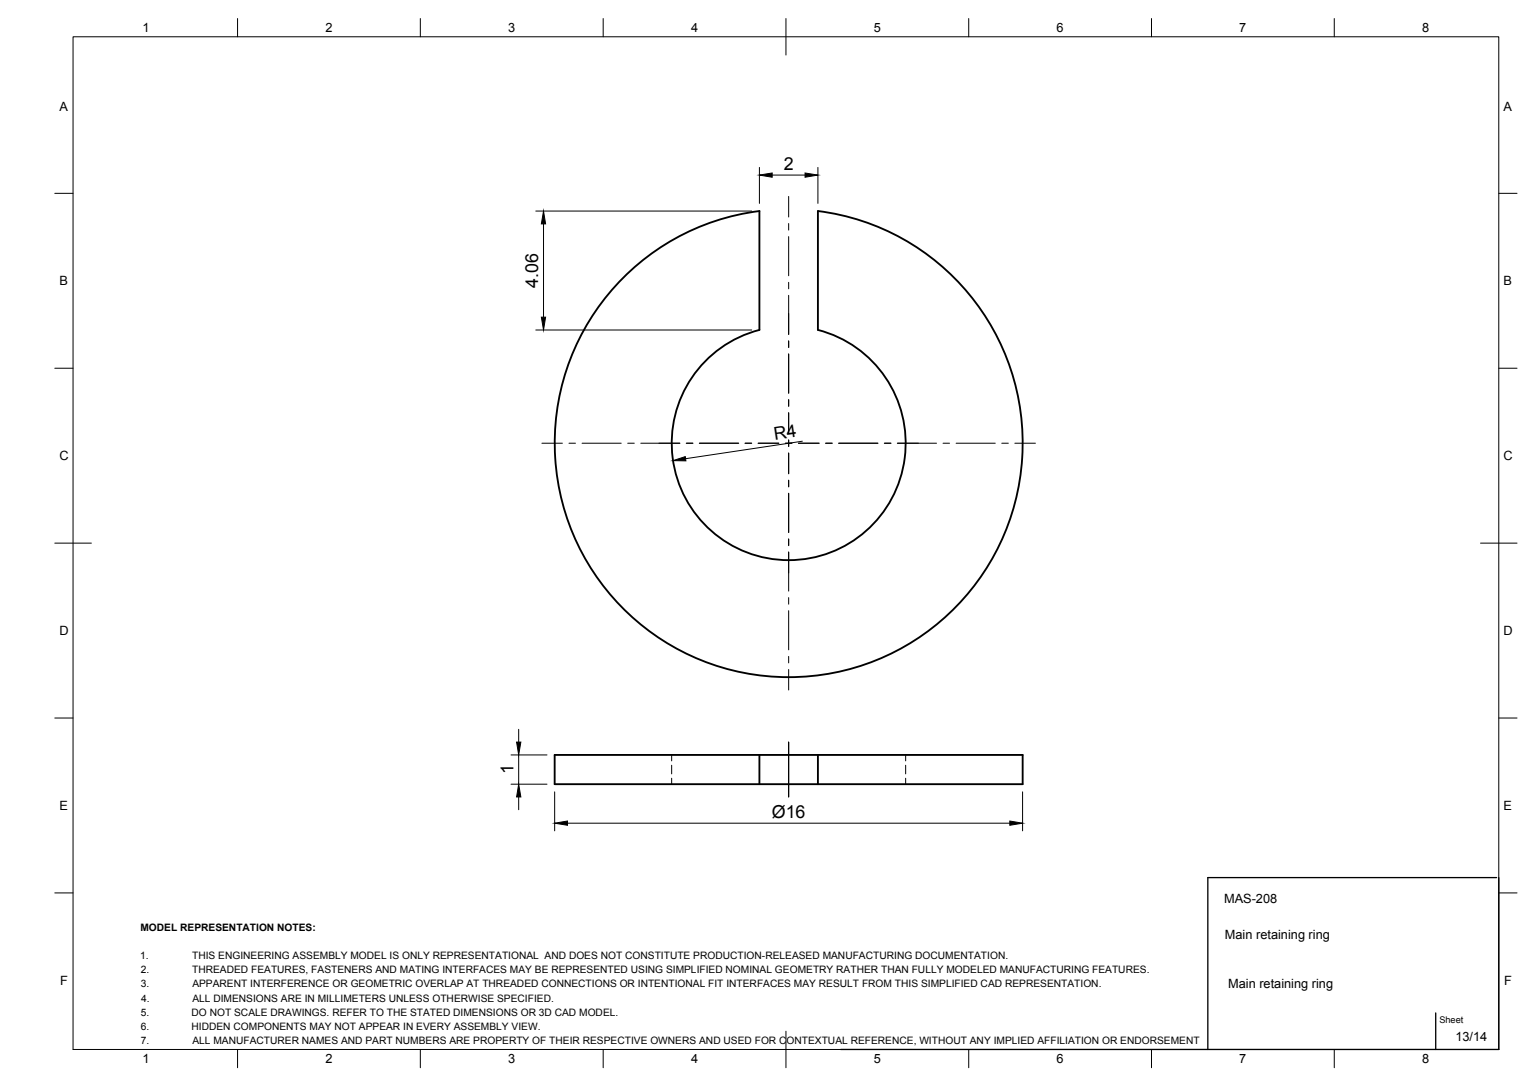
ISO-10303-21;
HEADER;
/* Generated by software containing ST-Developer
 * from STEP Tools, Inc. (www.steptools.com) 
 */

FILE_DESCRIPTION(
/* description */ ('Independent vertical20-tooth ratchet advance with repeated integral-c
ounterweight gravity pawls, swinging drive lever, bronze sleeves and f
ully retained axle stacks.18degpertooth. Native revolutes; geometric c
ycle checking rather than automatic contact/rolling dynamics. Gravity 
closing checked from actual pawl center of mass. Backplate/foot suppor
ts unit. Fits, torque, holding force, wear and life unassigned.'),
/* implementation_level */ '2;1');

FILE_NAME(
/* name */ 'Main retaining ring.step',
/* time_stamp */ '2026-11-09T06:25:53-08:00',
/* author */ (''),
/* organization */ (''),
/* preprocessor_version */ 'ST-DEVELOPER v20.2',
/* originating_system */ 'Autodesk Translation Framework v15.17.0.0',
/* authorisation */ '');

FILE_SCHEMA (('AUTOMOTIVE_DESIGN { 1 0 10303 214 3 1 1 }'));
ENDSEC;

DATA;
#10=MECHANICAL_DESIGN_GEOMETRIC_PRESENTATION_REPRESENTATION('',(#129),#4643);
#101=SHAPE_REPRESENTATION_RELATIONSHIP('SRR','None',#4706,#115);
#115=ADVANCED_BREP_SHAPE_REPRESENTATION('',(#143),#4635);
#129=STYLED_ITEM('',(#4783),#143);
#143=MANIFOLD_SOLID_BREP('Body1',#2665);
#269=PLANE('',#2979);
#270=PLANE('',#2980);
#271=PLANE('',#2981);
#272=PLANE('',#2988);
#403=FACE_OUTER_BOUND('',#581,.T.);
#404=FACE_OUTER_BOUND('',#582,.T.);
#405=FACE_OUTER_BOUND('',#583,.T.);
#406=FACE_OUTER_BOUND('',#584,.T.);
#407=FACE_OUTER_BOUND('',#585,.T.);
#408=FACE_OUTER_BOUND('',#586,.T.);
#581=EDGE_LOOP('',(#2269,#2270,#2271,#2272));
#582=EDGE_LOOP('',(#2273,#2274,#2275,#2276));
#583=EDGE_LOOP('',(#2277,#2278,#2279,#2280));
#584=EDGE_LOOP('',(#2281,#2282,#2283,#2284));
#585=EDGE_LOOP('',(#2285,#2286,#2287,#2288));
#586=EDGE_LOOP('',(#2289,#2290,#2291,#2292));
#833=LINE('',#4367,#1095);
#834=LINE('',#4369,#1096);
#835=LINE('',#4371,#1097);
#836=LINE('',#4372,#1098);
#837=LINE('',#4376,#1099);
#838=LINE('',#4378,#1100);
#839=LINE('',#4380,#1101);
#840=LINE('',#4381,#1102);
#1095=VECTOR('',#3581,10.);
#1096=VECTOR('',#3582,10.);
#1097=VECTOR('',#3583,10.);
#1098=VECTOR('',#3584,10.);
#1099=VECTOR('',#3587,10.);
#1100=VECTOR('',#3588,10.);
#1101=VECTOR('',#3589,10.);
#1102=VECTOR('',#3590,10.);
#1211=CIRCLE('',#2982,8.);
#1212=CIRCLE('',#2983,4.);
#1213=CIRCLE('',#2985,4.);
#1214=CIRCLE('',#2987,8.);
#1397=VERTEX_POINT('',#4365);
#1398=VERTEX_POINT('',#4366);
#1399=VERTEX_POINT('',#4368);
#1400=VERTEX_POINT('',#4370);
#1401=VERTEX_POINT('',#4374);
#1402=VERTEX_POINT('',#4375);
#1403=VERTEX_POINT('',#4377);
#1404=VERTEX_POINT('',#4379);
#1699=EDGE_CURVE('',#1397,#1398,#833,.T.);
#1700=EDGE_CURVE('',#1399,#1397,#834,.T.);
#1701=EDGE_CURVE('',#1400,#1399,#835,.T.);
#1702=EDGE_CURVE('',#1398,#1400,#836,.T.);
#1703=EDGE_CURVE('',#1401,#1402,#837,.T.);
#1704=EDGE_CURVE('',#1403,#1401,#838,.T.);
#1705=EDGE_CURVE('',#1404,#1403,#839,.T.);
#1706=EDGE_CURVE('',#1402,#1404,#840,.T.);
#1707=EDGE_CURVE('',#1399,#1404,#1211,.T.);
#1708=EDGE_CURVE('',#1402,#1397,#1212,.T.);
#1709=EDGE_CURVE('',#1401,#1398,#1213,.T.);
#1710=EDGE_CURVE('',#1400,#1403,#1214,.T.);
#2269=ORIENTED_EDGE('',*,*,#1699,.F.);
#2270=ORIENTED_EDGE('',*,*,#1700,.F.);
#2271=ORIENTED_EDGE('',*,*,#1701,.F.);
#2272=ORIENTED_EDGE('',*,*,#1702,.F.);
#2273=ORIENTED_EDGE('',*,*,#1703,.F.);
#2274=ORIENTED_EDGE('',*,*,#1704,.F.);
#2275=ORIENTED_EDGE('',*,*,#1705,.F.);
#2276=ORIENTED_EDGE('',*,*,#1706,.F.);
#2277=ORIENTED_EDGE('',*,*,#1706,.T.);
#2278=ORIENTED_EDGE('',*,*,#1707,.F.);
#2279=ORIENTED_EDGE('',*,*,#1700,.T.);
#2280=ORIENTED_EDGE('',*,*,#1708,.F.);
#2281=ORIENTED_EDGE('',*,*,#1703,.T.);
#2282=ORIENTED_EDGE('',*,*,#1708,.T.);
#2283=ORIENTED_EDGE('',*,*,#1699,.T.);
#2284=ORIENTED_EDGE('',*,*,#1709,.F.);
#2285=ORIENTED_EDGE('',*,*,#1705,.T.);
#2286=ORIENTED_EDGE('',*,*,#1710,.F.);
#2287=ORIENTED_EDGE('',*,*,#1701,.T.);
#2288=ORIENTED_EDGE('',*,*,#1707,.T.);
#2289=ORIENTED_EDGE('',*,*,#1704,.T.);
#2290=ORIENTED_EDGE('',*,*,#1709,.T.);
#2291=ORIENTED_EDGE('',*,*,#1702,.T.);
#2292=ORIENTED_EDGE('',*,*,#1710,.T.);
#2495=CYLINDRICAL_SURFACE('',#2984,4.);
#2496=CYLINDRICAL_SURFACE('',#2986,8.);
#2609=ADVANCED_FACE('',(#403),#269,.F.);
#2610=ADVANCED_FACE('',(#404),#270,.F.);
#2611=ADVANCED_FACE('',(#405),#271,.F.);
#2612=ADVANCED_FACE('',(#406),#2495,.F.);
#2613=ADVANCED_FACE('',(#407),#2496,.T.);
#2614=ADVANCED_FACE('',(#408),#272,.T.);
#2665=CLOSED_SHELL('',(#2609,#2610,#2611,#2612,#2613,#2614));
#2978=AXIS2_PLACEMENT_3D('',#4363,#3577,#3578);
#2979=AXIS2_PLACEMENT_3D('',#4364,#3579,#3580);
#2980=AXIS2_PLACEMENT_3D('',#4373,#3585,#3586);
#2981=AXIS2_PLACEMENT_3D('',#4382,#3591,#3592);
#2982=AXIS2_PLACEMENT_3D('',#4383,#3593,#3594);
#2983=AXIS2_PLACEMENT_3D('',#4384,#3595,#3596);
#2984=AXIS2_PLACEMENT_3D('',#4385,#3597,#3598);
#2985=AXIS2_PLACEMENT_3D('',#4386,#3599,#3600);
#2986=AXIS2_PLACEMENT_3D('',#4387,#3601,#3602);
#2987=AXIS2_PLACEMENT_3D('',#4388,#3603,#3604);
#2988=AXIS2_PLACEMENT_3D('',#4389,#3605,#3606);
#3577=DIRECTION('axis',(0.,0.,1.));
#3578=DIRECTION('refdir',(1.,0.,0.));
#3579=DIRECTION('center_axis',(-1.,0.,0.));
#3580=DIRECTION('ref_axis',(0.,1.,0.));
#3581=DIRECTION('',(0.,0.,1.));
#3582=DIRECTION('',(0.,-1.,0.));
#3583=DIRECTION('',(0.,0.,-1.));
#3584=DIRECTION('',(0.,1.,0.));
#3585=DIRECTION('center_axis',(1.,0.,0.));
#3586=DIRECTION('ref_axis',(0.,-1.,0.));
#3587=DIRECTION('',(0.,0.,-1.));
#3588=DIRECTION('',(0.,-1.,0.));
#3589=DIRECTION('',(0.,0.,1.));
#3590=DIRECTION('',(0.,1.,0.));
#3591=DIRECTION('center_axis',(0.,0.,1.));
#3592=DIRECTION('ref_axis',(1.,0.,0.));
#3593=DIRECTION('center_axis',(0.,0.,1.));
#3594=DIRECTION('ref_axis',(1.,0.,0.));
#3595=DIRECTION('center_axis',(0.,0.,-1.));
#3596=DIRECTION('ref_axis',(1.,0.,0.));
#3597=DIRECTION('center_axis',(0.,0.,1.));
#3598=DIRECTION('ref_axis',(6.12323399573677E-17,-1.,0.));
#3599=DIRECTION('center_axis',(0.,0.,-1.));
#3600=DIRECTION('ref_axis',(1.,0.,0.));
#3601=DIRECTION('center_axis',(0.,0.,1.));
#3602=DIRECTION('ref_axis',(6.12323399573677E-17,-1.,0.));
#3603=DIRECTION('center_axis',(0.,0.,1.));
#3604=DIRECTION('ref_axis',(1.,0.,0.));
#3605=DIRECTION('center_axis',(0.,0.,1.));
#3606=DIRECTION('ref_axis',(1.,0.,0.));
#4363=CARTESIAN_POINT('',(0.,0.,0.));
#4364=CARTESIAN_POINT('Origin',(-1.,0.,1.));
#4365=CARTESIAN_POINT('',(-1.,3.87298334620742,0.));
#4366=CARTESIAN_POINT('',(-1.,3.87298334620742,1.));
#4367=CARTESIAN_POINT('',(-1.,3.87298334620742,0.));
#4368=CARTESIAN_POINT('',(-1.,7.93725393319377,0.));
#4369=CARTESIAN_POINT('',(-1.,0.,0.));
#4370=CARTESIAN_POINT('',(-1.,7.93725393319377,1.));
#4371=CARTESIAN_POINT('',(-1.,7.93725393319377,0.));
#4372=CARTESIAN_POINT('',(-1.,0.,1.));
#4373=CARTESIAN_POINT('Origin',(1.,16.,1.));
#4374=CARTESIAN_POINT('',(1.,3.87298334620742,1.));
#4375=CARTESIAN_POINT('',(1.,3.87298334620742,0.));
#4376=CARTESIAN_POINT('',(1.,3.87298334620742,0.));
#4377=CARTESIAN_POINT('',(1.,7.93725393319377,1.));
#4378=CARTESIAN_POINT('',(1.,8.,1.));
#4379=CARTESIAN_POINT('',(1.,7.93725393319377,0.));
#4380=CARTESIAN_POINT('',(1.,7.93725393319377,0.));
#4381=CARTESIAN_POINT('',(1.,8.,0.));
#4382=CARTESIAN_POINT('Origin',(0.,0.,0.));
#4383=CARTESIAN_POINT('Origin',(0.,0.,0.));
#4384=CARTESIAN_POINT('Origin',(0.,0.,0.));
#4385=CARTESIAN_POINT('Origin',(0.,0.,0.));
#4386=CARTESIAN_POINT('Origin',(0.,0.,1.));
#4387=CARTESIAN_POINT('Origin',(0.,0.,0.));
#4388=CARTESIAN_POINT('Origin',(0.,0.,1.));
#4389=CARTESIAN_POINT('Origin',(0.,0.,1.));
#4619=UNCERTAINTY_MEASURE_WITH_UNIT(LENGTH_MEASURE(0.01),#4644,
'DISTANCE_ACCURACY_VALUE',
'Maximum model space distance between geometric entities at asserted c
onnectivities');
#4627=UNCERTAINTY_MEASURE_WITH_UNIT(LENGTH_MEASURE(0.01),#4644,
'DISTANCE_ACCURACY_VALUE',
'Maximum model space distance between geometric entities at asserted c
onnectivities');
#4635=(
GEOMETRIC_REPRESENTATION_CONTEXT(3)
GLOBAL_UNCERTAINTY_ASSIGNED_CONTEXT((#4619))
GLOBAL_UNIT_ASSIGNED_CONTEXT((#4644,#4646,#4647))
REPRESENTATION_CONTEXT('','3D')
);
#4643=(
GEOMETRIC_REPRESENTATION_CONTEXT(3)
GLOBAL_UNCERTAINTY_ASSIGNED_CONTEXT((#4627))
GLOBAL_UNIT_ASSIGNED_CONTEXT((#4644,#4646,#4647))
REPRESENTATION_CONTEXT('','3D')
);
#4644=(
LENGTH_UNIT()
NAMED_UNIT(*)
SI_UNIT(.MILLI.,.METRE.)
);
#4646=(
NAMED_UNIT(*)
PLANE_ANGLE_UNIT()
SI_UNIT($,.RADIAN.)
);
#4647=(
NAMED_UNIT(*)
SI_UNIT($,.STERADIAN.)
SOLID_ANGLE_UNIT()
);
#4655=SHAPE_DEFINITION_REPRESENTATION(#4670,#4706);
#4670=PRODUCT_DEFINITION_SHAPE('',$,#4722);
#4706=SHAPE_REPRESENTATION('',(#2978),#4635);
#4714=PRODUCT_DEFINITION_CONTEXT('part definition',#4761,'design');
#4722=PRODUCT_DEFINITION('Main retaining ring','Main retaining ring',#4737,
#4714);
#4737=PRODUCT_DEFINITION_FORMATION('',$,#4770);
#4761=APPLICATION_CONTEXT(
'Core Data for Automotive Mechanical Design Process');
#4762=PRODUCT_CONTEXT('part definition',#4761,'mechanical');
#4770=PRODUCT('Main retaining ring','Main retaining ring',$,(#4762));
#4783=PRESENTATION_STYLE_ASSIGNMENT((#4792));
#4792=SURFACE_STYLE_USAGE(.BOTH.,#4801);
#4801=SURFACE_SIDE_STYLE('',(#4810));
#4810=SURFACE_STYLE_FILL_AREA(#4819);
#4819=FILL_AREA_STYLE('Dark gray',(#4828));
#4828=FILL_AREA_STYLE_COLOUR('Dark gray',#4837);
#4837=COLOUR_RGB('Dark gray',0.250980392156863,0.282352941176471,0.32156862745098);
ENDSEC;
END-ISO-10303-21;
